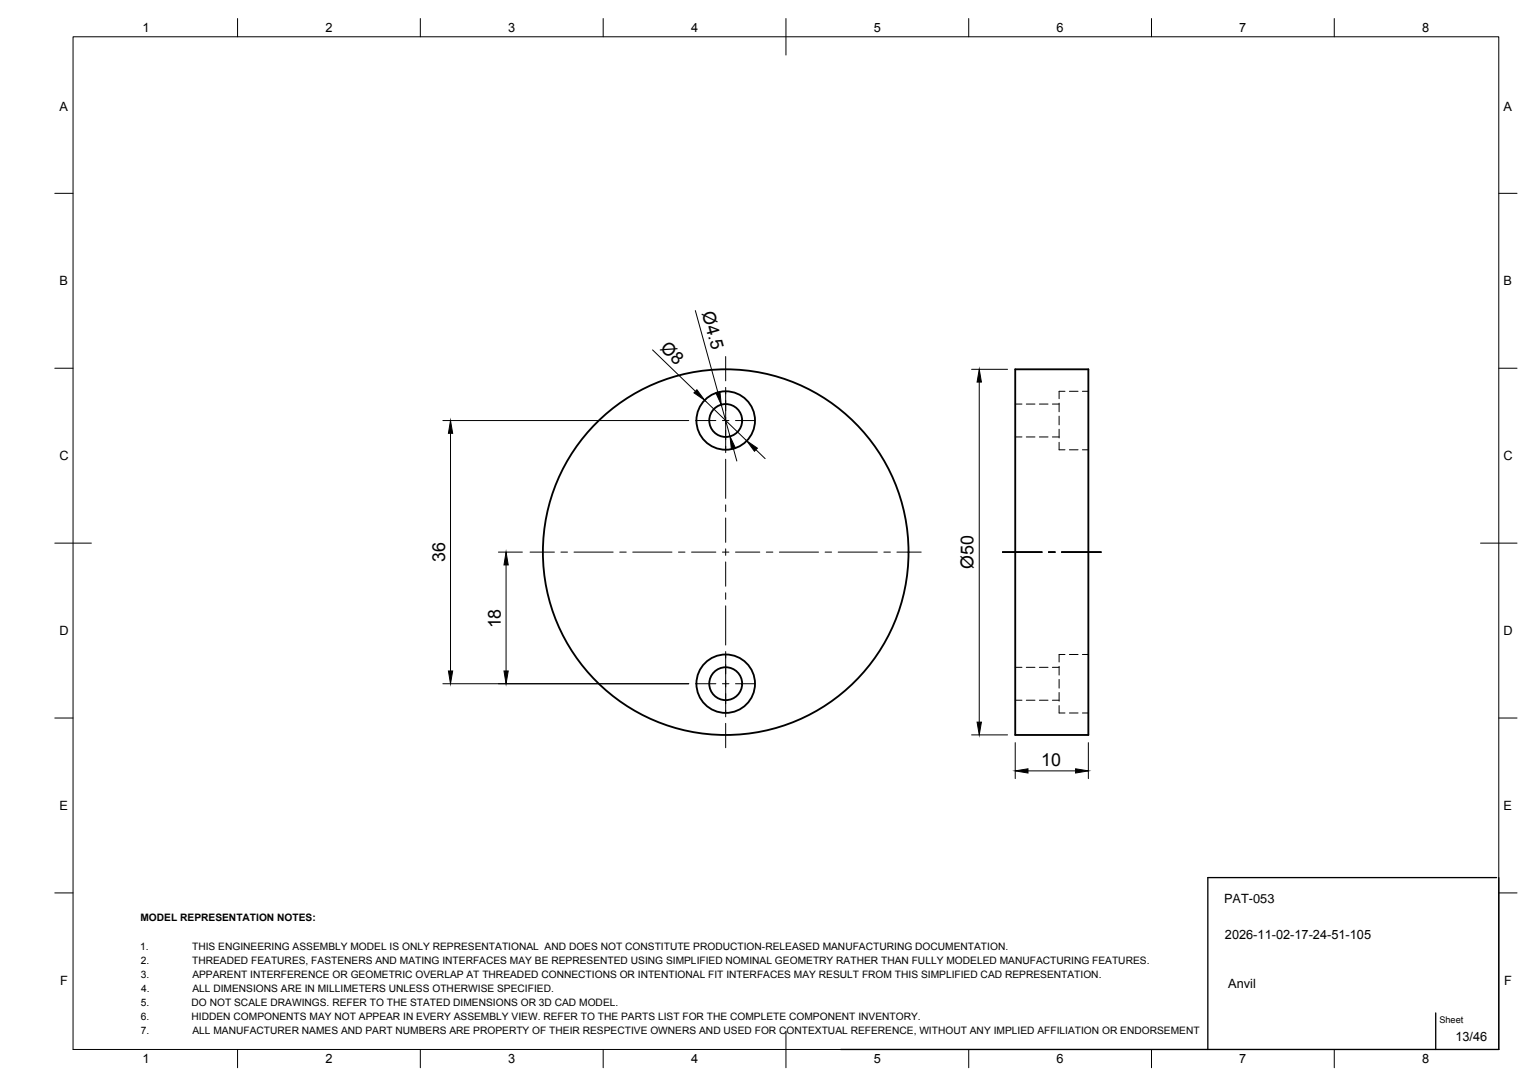
ISO-10303-21;
HEADER;
/* Generated by software containing ST-Developer
 * from STEP Tools, Inc. (www.steptools.com) 
 */

FILE_DESCRIPTION(
/* description */ ('Hand-operated arbor press'),
/* implementation_level */ '2;1');

FILE_NAME(
/* name */ 'Anvil.step',
/* time_stamp */ '2026-10-28T03:25:25-07:00',
/* author */ (''),
/* organization */ (''),
/* preprocessor_version */ 'ST-DEVELOPER v20.2',
/* originating_system */ 'Autodesk Translation Framework v15.17.0.0',
/* authorisation */ '');

FILE_SCHEMA (('AUTOMOTIVE_DESIGN { 1 0 10303 214 3 1 1 }'));
ENDSEC;

DATA;
#10=MECHANICAL_DESIGN_GEOMETRIC_PRESENTATION_REPRESENTATION('',(#594),#32751);
#510=SHAPE_REPRESENTATION_RELATIONSHIP('SRR','None',#32939,#552);
#552=ADVANCED_BREP_SHAPE_REPRESENTATION('',(#643),#32713);
#594=STYLED_ITEM('',(#33235),#643);
#643=MANIFOLD_SOLID_BREP('Body1',#12491);
#723=FACE_BOUND('',#2136,.T.);
#724=FACE_BOUND('',#2139,.T.);
#725=FACE_BOUND('',#2144,.T.);
#726=FACE_BOUND('',#2145,.T.);
#727=FACE_BOUND('',#2147,.T.);
#728=FACE_BOUND('',#2148,.T.);
#930=PLANE('',#13202);
#931=PLANE('',#13207);
#932=PLANE('',#13216);
#933=PLANE('',#13217);
#1410=FACE_OUTER_BOUND('',#2134,.T.);
#1411=FACE_OUTER_BOUND('',#2135,.T.);
#1412=FACE_OUTER_BOUND('',#2137,.T.);
#1413=FACE_OUTER_BOUND('',#2138,.T.);
#1414=FACE_OUTER_BOUND('',#2140,.T.);
#1415=FACE_OUTER_BOUND('',#2141,.T.);
#1416=FACE_OUTER_BOUND('',#2142,.T.);
#1417=FACE_OUTER_BOUND('',#2143,.T.);
#1418=FACE_OUTER_BOUND('',#2146,.T.);
#2134=EDGE_LOOP('',(#8888,#8889,#8890,#8891));
#2135=EDGE_LOOP('',(#8892));
#2136=EDGE_LOOP('',(#8893));
#2137=EDGE_LOOP('',(#8894,#8895,#8896,#8897));
#2138=EDGE_LOOP('',(#8898));
#2139=EDGE_LOOP('',(#8899));
#2140=EDGE_LOOP('',(#8900,#8901,#8902,#8903));
#2141=EDGE_LOOP('',(#8904,#8905,#8906,#8907));
#2142=EDGE_LOOP('',(#8908,#8909,#8910,#8911));
#2143=EDGE_LOOP('',(#8912));
#2144=EDGE_LOOP('',(#8913));
#2145=EDGE_LOOP('',(#8914));
#2146=EDGE_LOOP('',(#8915));
#2147=EDGE_LOOP('',(#8916));
#2148=EDGE_LOOP('',(#8917));
#3034=LINE('',#18240,#4205);
#3035=LINE('',#18249,#4206);
#3036=LINE('',#18257,#4207);
#3037=LINE('',#18261,#4208);
#3038=LINE('',#18266,#4209);
#4205=VECTOR('',#14769,0.4);
#4206=VECTOR('',#14780,0.4);
#4207=VECTOR('',#14791,0.225);
#4208=VECTOR('',#14796,0.225);
#4209=VECTOR('',#14801,2.5);
#5238=CIRCLE('',#13200,0.4);
#5239=CIRCLE('',#13201,0.4);
#5240=CIRCLE('',#13203,0.225);
#5241=CIRCLE('',#13205,0.4);
#5242=CIRCLE('',#13206,0.4);
#5243=CIRCLE('',#13208,0.225);
#5244=CIRCLE('',#13210,0.225);
#5245=CIRCLE('',#13212,0.225);
#5246=CIRCLE('',#13214,2.5);
#5247=CIRCLE('',#13215,2.5);
#5744=VERTEX_POINT('',#18237);
#5745=VERTEX_POINT('',#18239);
#5746=VERTEX_POINT('',#18243);
#5747=VERTEX_POINT('',#18246);
#5748=VERTEX_POINT('',#18248);
#5749=VERTEX_POINT('',#18252);
#5750=VERTEX_POINT('',#18255);
#5751=VERTEX_POINT('',#18259);
#5752=VERTEX_POINT('',#18263);
#5753=VERTEX_POINT('',#18265);
#6947=EDGE_CURVE('',#5744,#5744,#5238,.T.);
#6948=EDGE_CURVE('',#5744,#5745,#3034,.T.);
#6949=EDGE_CURVE('',#5745,#5745,#5239,.T.);
#6950=EDGE_CURVE('',#5746,#5746,#5240,.T.);
#6951=EDGE_CURVE('',#5747,#5747,#5241,.T.);
#6952=EDGE_CURVE('',#5747,#5748,#3035,.T.);
#6953=EDGE_CURVE('',#5748,#5748,#5242,.T.);
#6954=EDGE_CURVE('',#5749,#5749,#5243,.T.);
#6955=EDGE_CURVE('',#5750,#5750,#5244,.T.);
#6956=EDGE_CURVE('',#5750,#5746,#3036,.T.);
#6957=EDGE_CURVE('',#5751,#5751,#5245,.T.);
#6958=EDGE_CURVE('',#5751,#5749,#3037,.T.);
#6959=EDGE_CURVE('',#5752,#5752,#5246,.T.);
#6960=EDGE_CURVE('',#5752,#5753,#3038,.T.);
#6961=EDGE_CURVE('',#5753,#5753,#5247,.T.);
#8888=ORIENTED_EDGE('',*,*,#6947,.F.);
#8889=ORIENTED_EDGE('',*,*,#6948,.T.);
#8890=ORIENTED_EDGE('',*,*,#6949,.F.);
#8891=ORIENTED_EDGE('',*,*,#6948,.F.);
#8892=ORIENTED_EDGE('',*,*,#6947,.T.);
#8893=ORIENTED_EDGE('',*,*,#6950,.F.);
#8894=ORIENTED_EDGE('',*,*,#6951,.F.);
#8895=ORIENTED_EDGE('',*,*,#6952,.T.);
#8896=ORIENTED_EDGE('',*,*,#6953,.F.);
#8897=ORIENTED_EDGE('',*,*,#6952,.F.);
#8898=ORIENTED_EDGE('',*,*,#6951,.T.);
#8899=ORIENTED_EDGE('',*,*,#6954,.F.);
#8900=ORIENTED_EDGE('',*,*,#6955,.F.);
#8901=ORIENTED_EDGE('',*,*,#6956,.T.);
#8902=ORIENTED_EDGE('',*,*,#6950,.T.);
#8903=ORIENTED_EDGE('',*,*,#6956,.F.);
#8904=ORIENTED_EDGE('',*,*,#6957,.F.);
#8905=ORIENTED_EDGE('',*,*,#6958,.T.);
#8906=ORIENTED_EDGE('',*,*,#6954,.T.);
#8907=ORIENTED_EDGE('',*,*,#6958,.F.);
#8908=ORIENTED_EDGE('',*,*,#6959,.F.);
#8909=ORIENTED_EDGE('',*,*,#6960,.T.);
#8910=ORIENTED_EDGE('',*,*,#6961,.T.);
#8911=ORIENTED_EDGE('',*,*,#6960,.F.);
#8912=ORIENTED_EDGE('',*,*,#6959,.T.);
#8913=ORIENTED_EDGE('',*,*,#6949,.T.);
#8914=ORIENTED_EDGE('',*,*,#6953,.T.);
#8915=ORIENTED_EDGE('',*,*,#6961,.F.);
#8916=ORIENTED_EDGE('',*,*,#6955,.T.);
#8917=ORIENTED_EDGE('',*,*,#6957,.T.);
#11678=CYLINDRICAL_SURFACE('',#13199,0.4);
#11679=CYLINDRICAL_SURFACE('',#13204,0.4);
#11680=CYLINDRICAL_SURFACE('',#13209,0.225);
#11681=CYLINDRICAL_SURFACE('',#13211,0.225);
#11682=CYLINDRICAL_SURFACE('',#13213,2.5);
#11919=ADVANCED_FACE('',(#1410),#11678,.F.);
#11920=ADVANCED_FACE('',(#1411,#723),#930,.T.);
#11921=ADVANCED_FACE('',(#1412),#11679,.F.);
#11922=ADVANCED_FACE('',(#1413,#724),#931,.T.);
#11923=ADVANCED_FACE('',(#1414),#11680,.F.);
#11924=ADVANCED_FACE('',(#1415),#11681,.F.);
#11925=ADVANCED_FACE('',(#1416),#11682,.T.);
#11926=ADVANCED_FACE('',(#1417,#725,#726),#932,.T.);
#11927=ADVANCED_FACE('',(#1418,#727,#728),#933,.F.);
#12491=CLOSED_SHELL('',(#11919,#11920,#11921,#11922,#11923,#11924,#11925,
#11926,#11927));
#13198=AXIS2_PLACEMENT_3D('',#18235,#14763,#14764);
#13199=AXIS2_PLACEMENT_3D('',#18236,#14765,#14766);
#13200=AXIS2_PLACEMENT_3D('',#18238,#14767,#14768);
#13201=AXIS2_PLACEMENT_3D('',#18241,#14770,#14771);
#13202=AXIS2_PLACEMENT_3D('',#18242,#14772,#14773);
#13203=AXIS2_PLACEMENT_3D('',#18244,#14774,#14775);
#13204=AXIS2_PLACEMENT_3D('',#18245,#14776,#14777);
#13205=AXIS2_PLACEMENT_3D('',#18247,#14778,#14779);
#13206=AXIS2_PLACEMENT_3D('',#18250,#14781,#14782);
#13207=AXIS2_PLACEMENT_3D('',#18251,#14783,#14784);
#13208=AXIS2_PLACEMENT_3D('',#18253,#14785,#14786);
#13209=AXIS2_PLACEMENT_3D('',#18254,#14787,#14788);
#13210=AXIS2_PLACEMENT_3D('',#18256,#14789,#14790);
#13211=AXIS2_PLACEMENT_3D('',#18258,#14792,#14793);
#13212=AXIS2_PLACEMENT_3D('',#18260,#14794,#14795);
#13213=AXIS2_PLACEMENT_3D('',#18262,#14797,#14798);
#13214=AXIS2_PLACEMENT_3D('',#18264,#14799,#14800);
#13215=AXIS2_PLACEMENT_3D('',#18267,#14802,#14803);
#13216=AXIS2_PLACEMENT_3D('',#18268,#14804,#14805);
#13217=AXIS2_PLACEMENT_3D('',#18269,#14806,#14807);
#14763=DIRECTION('axis',(0.,0.,1.));
#14764=DIRECTION('refdir',(1.,0.,0.));
#14765=DIRECTION('center_axis',(0.,0.,1.));
#14766=DIRECTION('ref_axis',(1.,0.,0.));
#14767=DIRECTION('center_axis',(0.,0.,1.));
#14768=DIRECTION('ref_axis',(1.,0.,0.));
#14769=DIRECTION('',(0.,0.,1.));
#14770=DIRECTION('center_axis',(0.,0.,-1.));
#14771=DIRECTION('ref_axis',(1.,0.,0.));
#14772=DIRECTION('center_axis',(0.,0.,1.));
#14773=DIRECTION('ref_axis',(1.,0.,0.));
#14774=DIRECTION('center_axis',(0.,0.,1.));
#14775=DIRECTION('ref_axis',(1.,0.,0.));
#14776=DIRECTION('center_axis',(0.,0.,1.));
#14777=DIRECTION('ref_axis',(1.,0.,0.));
#14778=DIRECTION('center_axis',(0.,0.,1.));
#14779=DIRECTION('ref_axis',(1.,0.,0.));
#14780=DIRECTION('',(0.,0.,1.));
#14781=DIRECTION('center_axis',(0.,0.,-1.));
#14782=DIRECTION('ref_axis',(1.,0.,0.));
#14783=DIRECTION('center_axis',(0.,0.,1.));
#14784=DIRECTION('ref_axis',(1.,0.,0.));
#14785=DIRECTION('center_axis',(0.,0.,1.));
#14786=DIRECTION('ref_axis',(1.,0.,0.));
#14787=DIRECTION('center_axis',(0.,0.,1.));
#14788=DIRECTION('ref_axis',(1.,0.,0.));
#14789=DIRECTION('center_axis',(0.,0.,1.));
#14790=DIRECTION('ref_axis',(1.,0.,0.));
#14791=DIRECTION('',(0.,0.,1.));
#14792=DIRECTION('center_axis',(0.,0.,1.));
#14793=DIRECTION('ref_axis',(1.,0.,0.));
#14794=DIRECTION('center_axis',(0.,0.,1.));
#14795=DIRECTION('ref_axis',(1.,0.,0.));
#14796=DIRECTION('',(0.,0.,1.));
#14797=DIRECTION('center_axis',(0.,0.,1.));
#14798=DIRECTION('ref_axis',(1.,0.,0.));
#14799=DIRECTION('center_axis',(0.,0.,1.));
#14800=DIRECTION('ref_axis',(1.,0.,0.));
#14801=DIRECTION('',(0.,0.,-1.));
#14802=DIRECTION('center_axis',(0.,0.,1.));
#14803=DIRECTION('ref_axis',(1.,0.,0.));
#14804=DIRECTION('center_axis',(0.,0.,1.));
#14805=DIRECTION('ref_axis',(1.,0.,0.));
#14806=DIRECTION('center_axis',(0.,0.,1.));
#14807=DIRECTION('ref_axis',(1.,0.,0.));
#18235=CARTESIAN_POINT('',(0.,0.,0.));
#18236=CARTESIAN_POINT('Origin',(1.,-1.8,1.6));
#18237=CARTESIAN_POINT('',(0.6,-1.8,1.6));
#18238=CARTESIAN_POINT('Origin',(1.,-1.8,1.6));
#18239=CARTESIAN_POINT('',(0.6,-1.8,2.));
#18240=CARTESIAN_POINT('',(0.6,-1.8,1.6));
#18241=CARTESIAN_POINT('Origin',(1.,-1.8,2.));
#18242=CARTESIAN_POINT('Origin',(1.,-1.8,1.6));
#18243=CARTESIAN_POINT('',(0.775,-1.8,1.6));
#18244=CARTESIAN_POINT('Origin',(1.,-1.8,1.6));
#18245=CARTESIAN_POINT('Origin',(1.,1.8,1.6));
#18246=CARTESIAN_POINT('',(0.6,1.8,1.6));
#18247=CARTESIAN_POINT('Origin',(1.,1.8,1.6));
#18248=CARTESIAN_POINT('',(0.6,1.8,2.));
#18249=CARTESIAN_POINT('',(0.6,1.8,1.6));
#18250=CARTESIAN_POINT('Origin',(1.,1.8,2.));
#18251=CARTESIAN_POINT('Origin',(1.,1.8,1.6));
#18252=CARTESIAN_POINT('',(0.775,1.8,1.6));
#18253=CARTESIAN_POINT('Origin',(1.,1.8,1.6));
#18254=CARTESIAN_POINT('Origin',(1.,-1.8,0.9));
#18255=CARTESIAN_POINT('',(0.775,-1.8,1.));
#18256=CARTESIAN_POINT('Origin',(1.,-1.8,1.));
#18257=CARTESIAN_POINT('',(0.775,-1.8,0.9));
#18258=CARTESIAN_POINT('Origin',(1.,1.8,0.9));
#18259=CARTESIAN_POINT('',(0.775,1.8,1.));
#18260=CARTESIAN_POINT('Origin',(1.,1.8,1.));
#18261=CARTESIAN_POINT('',(0.775,1.8,0.9));
#18262=CARTESIAN_POINT('Origin',(1.,0.,1.));
#18263=CARTESIAN_POINT('',(-1.5,-3.06161699786838E-16,2.));
#18264=CARTESIAN_POINT('Origin',(1.,0.,2.));
#18265=CARTESIAN_POINT('',(-1.5,-3.06161699786838E-16,1.));
#18266=CARTESIAN_POINT('',(-1.5,-3.06161699786838E-16,1.));
#18267=CARTESIAN_POINT('Origin',(1.,0.,1.));
#18268=CARTESIAN_POINT('Origin',(1.,0.,2.));
#18269=CARTESIAN_POINT('Origin',(1.,0.,1.));
#32664=UNCERTAINTY_MEASURE_WITH_UNIT(LENGTH_MEASURE(0.001),#32752,
'DISTANCE_ACCURACY_VALUE',
'Maximum model space distance between geometric entities at asserted c
onnectivities');
#32702=UNCERTAINTY_MEASURE_WITH_UNIT(LENGTH_MEASURE(0.001),#32752,
'DISTANCE_ACCURACY_VALUE',
'Maximum model space distance between geometric entities at asserted c
onnectivities');
#32713=(
GEOMETRIC_REPRESENTATION_CONTEXT(3)
GLOBAL_UNCERTAINTY_ASSIGNED_CONTEXT((#32664))
GLOBAL_UNIT_ASSIGNED_CONTEXT((#32752,#32754,#32755))
REPRESENTATION_CONTEXT('','3D')
);
#32751=(
GEOMETRIC_REPRESENTATION_CONTEXT(3)
GLOBAL_UNCERTAINTY_ASSIGNED_CONTEXT((#32702))
GLOBAL_UNIT_ASSIGNED_CONTEXT((#32752,#32754,#32755))
REPRESENTATION_CONTEXT('','3D')
);
#32752=(
LENGTH_UNIT()
NAMED_UNIT(*)
SI_UNIT(.CENTI.,.METRE.)
);
#32754=(
NAMED_UNIT(*)
PLANE_ANGLE_UNIT()
SI_UNIT($,.RADIAN.)
);
#32755=(
NAMED_UNIT(*)
SI_UNIT($,.STERADIAN.)
SOLID_ANGLE_UNIT()
);
#32766=SHAPE_DEFINITION_REPRESENTATION(#32814,#32939);
#32814=PRODUCT_DEFINITION_SHAPE('',$,#32988);
#32939=SHAPE_REPRESENTATION('',(#13198),#32713);
#32977=PRODUCT_DEFINITION_CONTEXT('part definition',#33123,'design');
#32988=PRODUCT_DEFINITION('Anvil','Anvil',#33036,#32977);
#33036=PRODUCT_DEFINITION_FORMATION('',$,#33135);
#33123=APPLICATION_CONTEXT(
'Core Data for Automotive Mechanical Design Process');
#33124=PRODUCT_CONTEXT('part definition',#33123,'mechanical');
#33135=PRODUCT('Anvil','Anvil','Anvil',(#33124));
#33229=COLOUR_RGB('Sky Blue',0.24,0.69,0.87);
#33230=FILL_AREA_STYLE_COLOUR('',#33229);
#33231=FILL_AREA_STYLE('',(#33230));
#33232=SURFACE_STYLE_FILL_AREA(#33231);
#33233=SURFACE_SIDE_STYLE('',(#33232));
#33234=SURFACE_STYLE_USAGE(.BOTH.,#33233);
#33235=PRESENTATION_STYLE_ASSIGNMENT((#33234));
ENDSEC;
END-ISO-10303-21;
